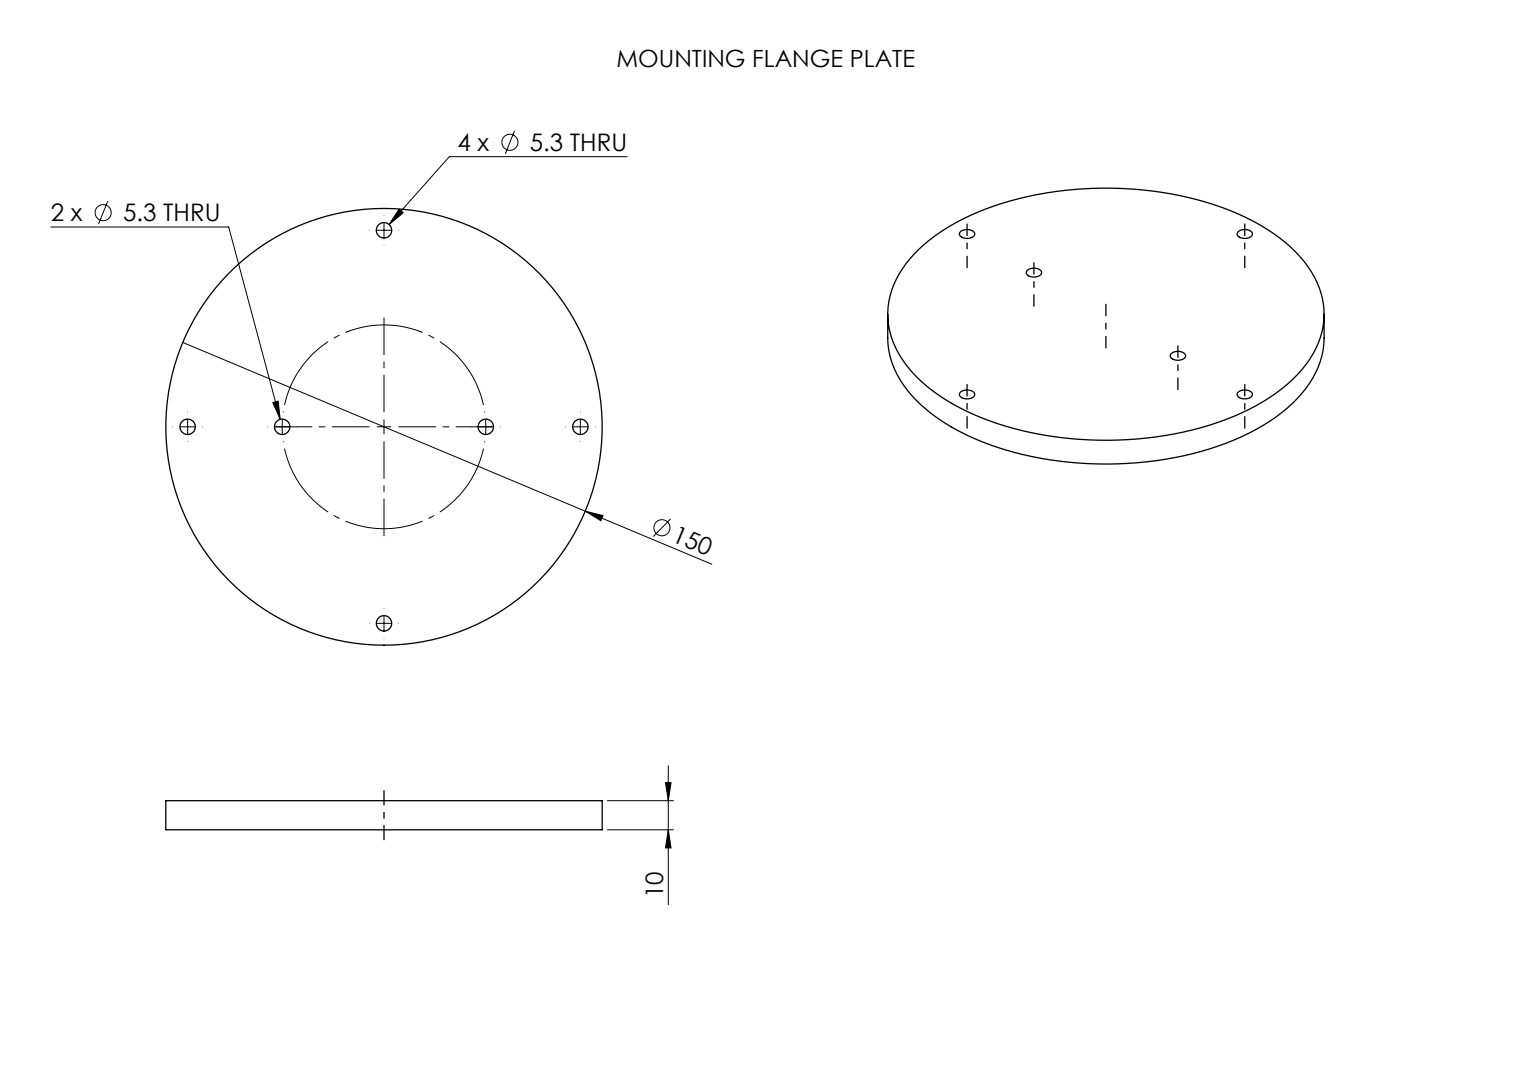
ISO-10303-21;
HEADER;
FILE_DESCRIPTION (('STEP AP214'),
    '1' );
FILE_NAME ('Mounting Flange Plate.step',
    '2026-10-08T13:56:24',
    ( '' ),
    ( '' ),
    'SwSTEP 2.0',
    'SolidWorks 2026',
    '' );
FILE_SCHEMA (( 'AUTOMOTIVE_DESIGN' ));
ENDSEC;

DATA;
#8=CARTESIAN_POINT ( 'NONE',  ( 0.000000000000000000, 50.00000000000000000, -75.00000000000004263 ) ) ;
#37=( NAMED_UNIT ( * ) PLANE_ANGLE_UNIT ( ) SI_UNIT ( $, .RADIAN. ) );
#45=LINE ( 'NONE', #8777, #8712 ) ;
#54=LINE ( 'NONE', #13437, #11247 ) ;
#74=VERTEX_POINT ( 'NONE', #3974 ) ;
#115=ORIENTED_EDGE ( 'NONE', *, *, #5097, .T. ) ;
#180=CIRCLE ( 'NONE', #13308, 2.649999999999985700 ) ;
#186=EDGE_CURVE ( 'NONE', #6462, #4993, #11776, .T. ) ;
#203=CIRCLE ( 'NONE', #1999, 2.649999999999992806 ) ;
#276=ADVANCED_FACE ( 'NONE', ( #4161 ), #12794, .F. ) ;
#288=ORIENTED_EDGE ( 'NONE', *, *, #2102, .T. ) ;
#323=ORIENTED_EDGE ( 'NONE', *, *, #1343, .T. ) ;
#330=ORIENTED_EDGE ( 'NONE', *, *, #5825, .T. ) ;
#378=ORIENTED_EDGE ( 'NONE', *, *, #14411, .F. ) ;
#384=DIRECTION ( 'NONE',  ( -0.000000000000000000, 1.000000000000000000, -0.000000000000000000 ) ) ;
#423=AXIS2_PLACEMENT_3D ( 'NONE', #12972, #1755, #11374 ) ;
#427=DIRECTION ( 'NONE',  ( 0.000000000000000000, 1.000000000000000000, 0.000000000000000000 ) ) ;
#439=ORIENTED_EDGE ( 'NONE', *, *, #14620, .F. ) ;
#514=CARTESIAN_POINT ( 'NONE',  ( 2.143131898507869826E-15, 40.00000000000000000, -64.85000000000002274 ) ) ;
#550=CYLINDRICAL_SURFACE ( 'NONE', #13850, 2.649999999999992806 ) ;
#577=ORIENTED_EDGE ( 'NONE', *, *, #4143, .F. ) ;
#602=CIRCLE ( 'NONE', #5747, 2.649999999999985700 ) ;
#613=DIRECTION ( 'NONE',  ( -0.000000000000000000, 1.000000000000000000, -0.000000000000000000 ) ) ;
#624=CARTESIAN_POINT ( 'NONE',  ( 67.49999999999931788, 50.00000000000000000, 2.081668171172168513E-14 ) ) ;
#663=ORIENTED_EDGE ( 'NONE', *, *, #8419, .F. ) ;
#681=AXIS2_PLACEMENT_3D ( 'NONE', #3435, #9655, #15746 ) ;
#778=DIRECTION ( 'NONE',  ( 0.000000000000000000, 0.000000000000000000, 1.000000000000000000 ) ) ;
#793=DIRECTION ( 'NONE',  ( 0.000000000000000000, 0.000000000000000000, 1.000000000000000000 ) ) ;
#841=DIRECTION ( 'NONE',  ( 0.000000000000000000, 0.000000000000000000, 1.000000000000000000 ) ) ;
#848=DIRECTION ( 'NONE',  ( 0.000000000000000000, 0.000000000000000000, 1.000000000000000000 ) ) ;
#921=CARTESIAN_POINT ( 'NONE',  ( -67.50000000000000000, 40.00000000000000000, 2.649999999999285816 ) ) ;
#934=EDGE_CURVE ( 'NONE', #2513, #13261, #602, .T. ) ;
#952=DIRECTION ( 'NONE',  ( 0.000000000000000000, 1.000000000000000000, 0.000000000000000000 ) ) ;
#988=MECHANICAL_DESIGN_GEOMETRIC_PRESENTATION_REPRESENTATION('',(#3323),#4608);
#1003=CARTESIAN_POINT ( 'NONE',  ( 35.00000000000000000, 50.00000000000000000, 2.649999999999985700 ) ) ;
#1012=DIRECTION ( 'NONE',  ( 0.000000000000000000, 0.000000000000000000, 1.000000000000000000 ) ) ;
#1025=ORIENTED_EDGE ( 'NONE', *, *, #5189, .F. ) ;
#1037=VERTEX_POINT ( 'NONE', #9465 ) ;
#1048=FACE_OUTER_BOUND ( 'NONE', #5833, .T. ) ;
#1071=( LENGTH_UNIT ( ) NAMED_UNIT ( * ) SI_UNIT ( .MILLI., .METRE. ) );
#1118=DIRECTION ( 'NONE',  ( -0.000000000000000000, 1.000000000000000000, -0.000000000000000000 ) ) ;
#1121=DIRECTION ( 'NONE',  ( 0.000000000000000000, -0.000000000000000000, 1.000000000000000000 ) ) ;
#1147=CIRCLE ( 'NONE', #10202, 2.649999999999985700 ) ;
#1152=ORIENTED_EDGE ( 'NONE', *, *, #13038, .F. ) ;
#1188=CIRCLE ( 'NONE', #14094, 2.649999999999985700 ) ;
#1194=EDGE_LOOP ( 'NONE', ( #577, #15095 ) ) ;
#1215=ORIENTED_EDGE ( 'NONE', *, *, #14990, .T. ) ;
#1221=VECTOR ( 'NONE', #2375, 1000.000000000000000 ) ;
#1240=CARTESIAN_POINT ( 'NONE',  ( 2.143131898507869826E-15, 50.00000000000000000, -67.50000000000000000 ) ) ;
#1299=ORIENTED_EDGE ( 'NONE', *, *, #3275, .F. ) ;
#1309=SHAPE_REPRESENTATION_RELATIONSHIP ( 'NONE' , 'NONE' ,  #3049, #6582 ) ;
#1338=DIRECTION ( 'NONE',  ( -0.000000000000000000, 1.000000000000000000, -0.000000000000000000 ) ) ;
#1343=EDGE_CURVE ( 'NONE', #4219, #74, #1876, .T. ) ;
#1369=LINE ( 'NONE', #10033, #13813 ) ;
#1412=EDGE_LOOP ( 'NONE', ( #9601, #5953, #4082, #1598 ) ) ;
#1417=AXIS2_PLACEMENT_3D ( 'NONE', #14635, #4617, #15541 ) ;
#1444=DIRECTION ( 'NONE',  ( -0.000000000000000000, 1.000000000000000000, -0.000000000000000000 ) ) ;
#1557=ADVANCED_FACE ( 'NONE', ( #1841 ), #4363, .F. ) ;
#1598=ORIENTED_EDGE ( 'NONE', *, *, #8419, .T. ) ;
#1624=CARTESIAN_POINT ( 'NONE',  ( -6.765421556309547668E-13, 40.00000000000000000, 67.49999999999930367 ) ) ;
#1658=ADVANCED_FACE ( 'NONE', ( #2550, #7189, #4907, #6041, #9667, #3612, #13379 ), #15756, .T. ) ;
#1679=ORIENTED_EDGE ( 'NONE', *, *, #6309, .F. ) ;
#1699=ORIENTED_EDGE ( 'NONE', *, *, #14620, .T. ) ;
#1709=AXIS2_PLACEMENT_3D ( 'NONE', #7658, #12787, #5294 ) ;
#1711=CARTESIAN_POINT ( 'NONE',  ( 35.00000000000000000, 50.00000000000000000, 2.649999999999992806 ) ) ;
#1726=CYLINDRICAL_SURFACE ( 'NONE', #14159, 2.649999999999992806 ) ;
#1755=DIRECTION ( 'NONE',  ( 0.000000000000000000, 1.000000000000000000, 0.000000000000000000 ) ) ;
#1806=DIRECTION ( 'NONE',  ( 0.000000000000000000, 0.000000000000000000, 1.000000000000000000 ) ) ;
#1841=FACE_OUTER_BOUND ( 'NONE', #15839, .T. ) ;
#1866=AXIS2_PLACEMENT_3D ( 'NONE', #14603, #3524, #3687 ) ;
#1876=CIRCLE ( 'NONE', #3686, 2.649999999999985700 ) ;
#1896=CARTESIAN_POINT ( 'NONE',  ( 35.00000000000000000, 40.00000000000000000, 0.000000000000000000 ) ) ;
#1910=EDGE_LOOP ( 'NONE', ( #3150, #8237 ) ) ;
#1982=VECTOR ( 'NONE', #15334, 1000.000000000000000 ) ;
#1999=AXIS2_PLACEMENT_3D ( 'NONE', #10864, #15807, #4723 ) ;
#2071=VERTEX_POINT ( 'NONE', #4724 ) ;
#2102=EDGE_CURVE ( 'NONE', #12678, #12016, #8834, .T. ) ;
#2181=DIRECTION ( 'NONE',  ( -0.000000000000000000, 1.000000000000000000, -0.000000000000000000 ) ) ;
#2199=( LENGTH_UNIT ( ) NAMED_UNIT ( * ) SI_UNIT ( .MILLI., .METRE. ) );
#2202=AXIS2_PLACEMENT_3D ( 'NONE', #14543, #3463, #3788 ) ;
#2204=ORIENTED_EDGE ( 'NONE', *, *, #4643, .T. ) ;
#2260=CARTESIAN_POINT ( 'NONE',  ( 35.00000000000000000, 40.00000000000000000, 0.000000000000000000 ) ) ;
#2281=EDGE_CURVE ( 'NONE', #15345, #10675, #14755, .T. ) ;
#2289=( NAMED_UNIT ( * ) PLANE_ANGLE_UNIT ( ) SI_UNIT ( $, .RADIAN. ) );
#2375=DIRECTION ( 'NONE',  ( -0.000000000000000000, -1.000000000000000000, -0.000000000000000000 ) ) ;
#2386=CARTESIAN_POINT ( 'NONE',  ( -67.50000000000000000, 50.00000000000000000, 2.649999999999278710 ) ) ;
#2455=ORIENTED_EDGE ( 'NONE', *, *, #8323, .T. ) ;
#2512=( LENGTH_UNIT ( ) NAMED_UNIT ( * ) SI_UNIT ( .MILLI., .METRE. ) );
#2513=VERTEX_POINT ( 'NONE', #13646 ) ;
#2534=ORIENTED_EDGE ( 'NONE', *, *, #8630, .F. ) ;
#2537=CARTESIAN_POINT ( 'NONE',  ( -35.00000000000000000, 50.00000000000000000, -2.649999999999992806 ) ) ;
#2550=FACE_BOUND ( 'NONE', #13651, .T. ) ;
#2561=EDGE_LOOP ( 'NONE', ( #1299, #2455, #1699, #1152 ) ) ;
#2598=( NAMED_UNIT ( * ) SI_UNIT ( $, .STERADIAN. ) SOLID_ANGLE_UNIT ( ) );
#2611=DIRECTION ( 'NONE',  ( -0.000000000000000000, 1.000000000000000000, -0.000000000000000000 ) ) ;
#2689=DIRECTION ( 'NONE',  ( 0.000000000000000000, 0.000000000000000000, 1.000000000000000000 ) ) ;
#2703=ORIENTED_EDGE ( 'NONE', *, *, #11988, .F. ) ;
#2726=DIRECTION ( 'NONE',  ( 0.000000000000000000, 1.000000000000000000, 0.000000000000000000 ) ) ;
#2738=DIRECTION ( 'NONE',  ( -0.000000000000000000, 1.000000000000000000, -0.000000000000000000 ) ) ;
#2811=ORIENTED_EDGE ( 'NONE', *, *, #6309, .T. ) ;
#2835=ORIENTED_EDGE ( 'NONE', *, *, #5189, .T. ) ;
#2841=DIRECTION ( 'NONE',  ( -0.000000000000000000, 1.000000000000000000, -0.000000000000000000 ) ) ;
#2873=APPLICATION_CONTEXT ( 'automotive_design' ) ;
#2874=FACE_OUTER_BOUND ( 'NONE', #3579, .T. ) ;
#2960=CYLINDRICAL_SURFACE ( 'NONE', #681, 75.00000000000004263 ) ;
#3021=VECTOR ( 'NONE', #13757, 1000.000000000000000 ) ;
#3049=SHAPE_REPRESENTATION ( 'Mounting Flange Plate', ( #3223 ), #15373 ) ;
#3055=ORIENTED_EDGE ( 'NONE', *, *, #4930, .F. ) ;
#3118=VERTEX_POINT ( 'NONE', #10334 ) ;
#3138=CARTESIAN_POINT ( 'NONE',  ( 67.49999999999931788, 40.00000000000000000, 2.081668171172168513E-14 ) ) ;
#3141=DIRECTION ( 'NONE',  ( 0.000000000000000000, 0.000000000000000000, 1.000000000000000000 ) ) ;
#3150=ORIENTED_EDGE ( 'NONE', *, *, #15289, .T. ) ;
#3191=VERTEX_POINT ( 'NONE', #5708 ) ;
#3223=AXIS2_PLACEMENT_3D ( 'NONE', #11897, #11972, #4638 ) ;
#3248=AXIS2_PLACEMENT_3D ( 'NONE', #15818, #3291, #793 ) ;
#3253=AXIS2_PLACEMENT_3D ( 'NONE', #3138, #8007, #14453 ) ;
#3266=CARTESIAN_POINT ( 'NONE',  ( -35.00000000000000000, 50.00000000000000000, 2.649999999999985700 ) ) ;
#3270=CYLINDRICAL_SURFACE ( 'NONE', #6972, 2.649999999999985700 ) ;
#3275=EDGE_CURVE ( 'NONE', #10300, #9472, #15960, .T. ) ;
#3291=DIRECTION ( 'NONE',  ( -0.000000000000000000, 1.000000000000000000, -0.000000000000000000 ) ) ;
#3323=STYLED_ITEM ( 'NONE', ( #14492 ), #9475 ) ;
#3435=CARTESIAN_POINT ( 'NONE',  ( 0.000000000000000000, 50.00000000000000000, 0.000000000000000000 ) ) ;
#3463=DIRECTION ( 'NONE',  ( -0.000000000000000000, 1.000000000000000000, -0.000000000000000000 ) ) ;
#3472=CIRCLE ( 'NONE', #10961, 75.00000000000004263 ) ;
#3524=DIRECTION ( 'NONE',  ( 0.000000000000000000, 1.000000000000000000, 0.000000000000000000 ) ) ;
#3543=CARTESIAN_POINT ( 'NONE',  ( -67.50000000000000000, 50.00000000000000000, 2.649999999999285816 ) ) ;
#3579=EDGE_LOOP ( 'NONE', ( #10493, #4203, #6813, #9254 ) ) ;
#3580=CARTESIAN_POINT ( 'NONE',  ( -6.765421556309547668E-13, 50.00000000000000000, 70.14999999999929514 ) ) ;
#3609=APPLICATION_CONTEXT ( 'automotive_design' ) ;
#3612=FACE_BOUND ( 'NONE', #11613, .T. ) ;
#3641=CARTESIAN_POINT ( 'NONE',  ( 9.184850993605153466E-15, 50.00000000000000000, 75.00000000000004263 ) ) ;
#3651=AXIS2_PLACEMENT_3D ( 'NONE', #2260, #10529, #9467 ) ;
#3657=SURFACE_STYLE_FILL_AREA ( #13668 ) ;
#3686=AXIS2_PLACEMENT_3D ( 'NONE', #6471, #1444, #10349 ) ;
#3687=DIRECTION ( 'NONE',  ( 0.000000000000000000, -0.000000000000000000, 1.000000000000000000 ) ) ;
#3703=ORIENTED_EDGE ( 'NONE', *, *, #14672, .F. ) ;
#3706=FACE_BOUND ( 'NONE', #13137, .T. ) ;
#3732=SURFACE_SIDE_STYLE ('',( #3657 ) ) ;
#3745=DIRECTION ( 'NONE',  ( -0.000000000000000000, 1.000000000000000000, -0.000000000000000000 ) ) ;
#3788=DIRECTION ( 'NONE',  ( 0.000000000000000000, 0.000000000000000000, 1.000000000000000000 ) ) ;
#3791=PLANE ( 'NONE',  #15961 ) ;
#3795=ADVANCED_FACE ( 'NONE', ( #12612 ), #6330, .F. ) ;
#3821=FILL_AREA_STYLE_COLOUR ( '', #6625 ) ;
#3898=DIRECTION ( 'NONE',  ( 0.000000000000000000, 1.000000000000000000, 0.000000000000000000 ) ) ;
#3923=DIRECTION ( 'NONE',  ( 0.000000000000000000, 0.000000000000000000, 1.000000000000000000 ) ) ;
#3964=CARTESIAN_POINT ( 'NONE',  ( 0.000000000000000000, 50.00000000000000000, 0.000000000000000000 ) ) ;
#3974=CARTESIAN_POINT ( 'NONE',  ( 2.143131898507869826E-15, 50.00000000000000000, -64.85000000000002274 ) ) ;
#3981=CARTESIAN_POINT ( 'NONE',  ( 67.49999999999931788, 50.00000000000000000, 2.650000000000013678 ) ) ;
#4019=EDGE_CURVE ( 'NONE', #10675, #15938, #5597, .T. ) ;
#4023=CIRCLE ( 'NONE', #423, 2.649999999999992806 ) ;
#4030=CARTESIAN_POINT ( 'NONE',  ( -67.50000000000000000, 50.00000000000000000, -7.070249711157346244E-13 ) ) ;
#4041=CIRCLE ( 'NONE', #9713, 2.649999999999985700 ) ;
#4082=ORIENTED_EDGE ( 'NONE', *, *, #13038, .T. ) ;
#4087=DIRECTION ( 'NONE',  ( 0.000000000000000000, 0.000000000000000000, 1.000000000000000000 ) ) ;
#4122=ORIENTED_EDGE ( 'NONE', *, *, #4947, .F. ) ;
#4143=EDGE_CURVE ( 'NONE', #2071, #14412, #180, .T. ) ;
#4161=FACE_OUTER_BOUND ( 'NONE', #10744, .T. ) ;
#4203=ORIENTED_EDGE ( 'NONE', *, *, #15548, .T. ) ;
#4219=VERTEX_POINT ( 'NONE', #4478 ) ;
#4247=DIRECTION ( 'NONE',  ( 0.000000000000000000, 0.000000000000000000, 1.000000000000000000 ) ) ;
#4259=ORIENTED_EDGE ( 'NONE', *, *, #186, .F. ) ;
#4335=CIRCLE ( 'NONE', #10006, 2.649999999999985700 ) ;
#4342=CARTESIAN_POINT ( 'NONE',  ( 35.00000000000000000, 50.00000000000000000, -2.649999999999992806 ) ) ;
#4363=CYLINDRICAL_SURFACE ( 'NONE', #7560, 2.649999999999985700 ) ;
#4440=VERTEX_POINT ( 'NONE', #2386 ) ;
#4443=ADVANCED_FACE ( 'NONE', ( #2874 ), #11200, .F. ) ;
#4450=ORIENTED_EDGE ( 'NONE', *, *, #7947, .T. ) ;
#4478=CARTESIAN_POINT ( 'NONE',  ( 2.467663300281918126E-15, 50.00000000000000000, -70.14999999999999147 ) ) ;
#4560=FACE_OUTER_BOUND ( 'NONE', #10471, .T. ) ;
#4569=VECTOR ( 'NONE', #14181, 1000.000000000000000 ) ;
#4595=LINE ( 'NONE', #14384, #1221 ) ;
#4607=VECTOR ( 'NONE', #12069, 1000.000000000000000 ) ;
#4608=( GEOMETRIC_REPRESENTATION_CONTEXT ( 3 ) GLOBAL_UNCERTAINTY_ASSIGNED_CONTEXT ( ( #14034 ) ) GLOBAL_UNIT_ASSIGNED_CONTEXT ( ( #2199, #15793, #10932 ) ) REPRESENTATION_CONTEXT ( 'NONE', 'WORKASPACE' ) );
#4617=DIRECTION ( 'NONE',  ( -0.000000000000000000, 1.000000000000000000, -0.000000000000000000 ) ) ;
#4638=DIRECTION ( 'NONE',  ( 1.000000000000000000, 0.000000000000000000, 0.000000000000000000 ) ) ;
#4643=EDGE_CURVE ( 'NONE', #6800, #6071, #9114, .T. ) ;
#4645=EDGE_LOOP ( 'NONE', ( #7116, #4799, #13900, #5382 ) ) ;
#4661=ADVANCED_FACE ( 'NONE', ( #13042 ), #550, .F. ) ;
#4694=ORIENTED_EDGE ( 'NONE', *, *, #4947, .T. ) ;
#4723=DIRECTION ( 'NONE',  ( 0.000000000000000000, 0.000000000000000000, 1.000000000000000000 ) ) ;
#4724=CARTESIAN_POINT ( 'NONE',  ( -6.765421556309547668E-13, 50.00000000000000000, 70.14999999999929514 ) ) ;
#4726=CARTESIAN_POINT ( 'NONE',  ( 2.467663300281917732E-15, 50.00000000000000000, -70.14999999999999147 ) ) ;
#4763=LINE ( 'NONE', #3543, #11243 ) ;
#4772=DIRECTION ( 'NONE',  ( 0.000000000000000000, 0.000000000000000000, 1.000000000000000000 ) ) ;
#4799=ORIENTED_EDGE ( 'NONE', *, *, #5413, .T. ) ;
#4821=EDGE_CURVE ( 'NONE', #3191, #6800, #5082, .T. ) ;
#4861=DIRECTION ( 'NONE',  ( -0.000000000000000000, 1.000000000000000000, -0.000000000000000000 ) ) ;
#4864=EDGE_LOOP ( 'NONE', ( #8155, #13074, #2811, #5258 ) ) ;
#4881=CARTESIAN_POINT ( 'NONE',  ( 9.184850993605153466E-15, 40.00000000000000000, 75.00000000000004263 ) ) ;
#4907=FACE_BOUND ( 'NONE', #8075, .T. ) ;
#4921=CARTESIAN_POINT ( 'NONE',  ( 67.49999999999931788, 50.00000000000000000, 2.650000000000006573 ) ) ;
#4923=EDGE_LOOP ( 'NONE', ( #8098, #8858 ) ) ;
#4930=EDGE_CURVE ( 'NONE', #6800, #3191, #203, .T. ) ;
#4947=EDGE_CURVE ( 'NONE', #74, #4219, #10273, .T. ) ;
#4950=LINE ( 'NONE', #3580, #7713 ) ;
#4993=VERTEX_POINT ( 'NONE', #14823 ) ;
#5029=( GEOMETRIC_REPRESENTATION_CONTEXT ( 3 ) GLOBAL_UNCERTAINTY_ASSIGNED_CONTEXT ( ( #12385 ) ) GLOBAL_UNIT_ASSIGNED_CONTEXT ( ( #2512, #2289, #2598 ) ) REPRESENTATION_CONTEXT ( 'NONE', 'WORKASPACE' ) );
#5044=DIRECTION ( 'NONE',  ( -0.000000000000000000, 1.000000000000000000, -0.000000000000000000 ) ) ;
#5062=EDGE_CURVE ( 'NONE', #12678, #74, #45, .T. ) ;
#5082=CIRCLE ( 'NONE', #8970, 2.649999999999992806 ) ;
#5097=EDGE_CURVE ( 'NONE', #6462, #11470, #13678, .T. ) ;
#5107=AXIS2_PLACEMENT_3D ( 'NONE', #10299, #2841, #9003 ) ;
#5122=CARTESIAN_POINT ( 'NONE',  ( 35.00000000000000000, 40.00000000000000000, 2.649999999999992806 ) ) ;
#5134=CARTESIAN_POINT ( 'NONE',  ( -35.00000000000000000, 50.00000000000000000, 0.000000000000000000 ) ) ;
#5189=EDGE_CURVE ( 'NONE', #9703, #1037, #12700, .T. ) ;
#5235=ORIENTED_EDGE ( 'NONE', *, *, #14818, .T. ) ;
#5258=ORIENTED_EDGE ( 'NONE', *, *, #4143, .T. ) ;
#5294=DIRECTION ( 'NONE',  ( 0.000000000000000000, 0.000000000000000000, 1.000000000000000000 ) ) ;
#5364=AXIS2_PLACEMENT_3D ( 'NONE', #1240, #3745, #2689 ) ;
#5382=ORIENTED_EDGE ( 'NONE', *, *, #4019, .F. ) ;
#5413=EDGE_CURVE ( 'NONE', #15345, #3118, #5551, .T. ) ;
#5432=DIRECTION ( 'NONE',  ( 0.000000000000000000, 0.000000000000000000, -1.000000000000000000 ) ) ;
#5442=ORIENTED_EDGE ( 'NONE', *, *, #14990, .F. ) ;
#5454=CARTESIAN_POINT ( 'NONE',  ( -67.50000000000000000, 50.00000000000000000, -7.070249711157346244E-13 ) ) ;
#5551=LINE ( 'NONE', #4342, #6910 ) ;
#5597=LINE ( 'NONE', #1711, #10011 ) ;
#5704=DIRECTION ( 'NONE',  ( -0.000000000000000000, 1.000000000000000000, -0.000000000000000000 ) ) ;
#5708=CARTESIAN_POINT ( 'NONE',  ( -35.00000000000000000, 40.00000000000000000, -2.649999999999992806 ) ) ;
#5747=AXIS2_PLACEMENT_3D ( 'NONE', #1624, #427, #15219 ) ;
#5766=CARTESIAN_POINT ( 'NONE',  ( -6.765421556309547668E-13, 50.00000000000000000, 67.49999999999930367 ) ) ;
#5768=ORIENTED_EDGE ( 'NONE', *, *, #14393, .F. ) ;
#5796=CIRCLE ( 'NONE', #14833, 2.649999999999992806 ) ;
#5825=EDGE_CURVE ( 'NONE', #14592, #10616, #4595, .T. ) ;
#5833=EDGE_LOOP ( 'NONE', ( #14308, #2703 ) ) ;
#5859=AXIS2_PLACEMENT_3D ( 'NONE', #3964, #10118, #5432 ) ;
#5865=LINE ( 'NONE', #4726, #4607 ) ;
#5895=AXIS2_PLACEMENT_3D ( 'NONE', #8233, #8070, #13129 ) ;
#5920=ORIENTED_EDGE ( 'NONE', *, *, #14818, .F. ) ;
#5935=EDGE_LOOP ( 'NONE', ( #12559, #8528 ) ) ;
#5936=DIRECTION ( 'NONE',  ( -0.000000000000000000, 1.000000000000000000, -0.000000000000000000 ) ) ;
#5953=ORIENTED_EDGE ( 'NONE', *, *, #15289, .F. ) ;
#5980=DIRECTION ( 'NONE',  ( 0.000000000000000000, 0.000000000000000000, 1.000000000000000000 ) ) ;
#6009=PRODUCT_DEFINITION ( 'UNKNOWN', '', #6905, #6432 ) ;
#6041=FACE_BOUND ( 'NONE', #8449, .T. ) ;
#6059=CARTESIAN_POINT ( 'NONE',  ( -6.765421556309547668E-13, 50.00000000000000000, 67.49999999999930367 ) ) ;
#6071=VERTEX_POINT ( 'NONE', #3266 ) ;
#6113=ORIENTED_EDGE ( 'NONE', *, *, #11650, .T. ) ;
#6229=FACE_BOUND ( 'NONE', #11318, .T. ) ;
#6309=EDGE_CURVE ( 'NONE', #2513, #2071, #4950, .T. ) ;
#6312=DIRECTION ( 'NONE',  ( -0.000000000000000000, 1.000000000000000000, -0.000000000000000000 ) ) ;
#6330=CYLINDRICAL_SURFACE ( 'NONE', #5107, 2.649999999999985700 ) ;
#6337=DIRECTION ( 'NONE',  ( 0.000000000000000000, 0.000000000000000000, 1.000000000000000000 ) ) ;
#6355=LINE ( 'NONE', #2537, #15909 ) ;
#6398=EDGE_LOOP ( 'NONE', ( #13187, #3055, #2204, #4450 ) ) ;
#6407=FACE_OUTER_BOUND ( 'NONE', #15268, .T. ) ;
#6432=PRODUCT_DEFINITION_CONTEXT ( 'detailed design', #3609, 'design' ) ;
#6462=VERTEX_POINT ( 'NONE', #9960 ) ;
#6471=CARTESIAN_POINT ( 'NONE',  ( 2.143131898507869826E-15, 50.00000000000000000, -67.50000000000000000 ) ) ;
#6562=ADVANCED_FACE ( 'NONE', ( #9777, #6229, #3706, #9929, #12352, #7209, #1048 ), #3791, .F. ) ;
#6582=ADVANCED_BREP_SHAPE_REPRESENTATION ( '', ( #9475, #3223 ), #15373 ) ;
#6625=COLOUR_RGB ( '', 0.09019608, 0.27058824, 0.51372549) ;
#6687=EDGE_LOOP ( 'NONE', ( #10153, #13602, #7741, #4694 ) ) ;
#6710=DIRECTION ( 'NONE',  ( 0.000000000000000000, 0.000000000000000000, 1.000000000000000000 ) ) ;
#6800=VERTEX_POINT ( 'NONE', #11106 ) ;
#6813=ORIENTED_EDGE ( 'NONE', *, *, #12208, .T. ) ;
#6905=PRODUCT_DEFINITION_FORMATION_WITH_SPECIFIED_SOURCE ( 'ANY', '', #8502, .NOT_KNOWN. ) ;
#6910=VECTOR ( 'NONE', #10576, 1000.000000000000000 ) ;
#6972=AXIS2_PLACEMENT_3D ( 'NONE', #15489, #5936, #848 ) ;
#7036=CARTESIAN_POINT ( 'NONE',  ( 0.000000000000000000, 50.00000000000000000, 0.000000000000000000 ) ) ;
#7067=PRODUCT_DEFINITION_SHAPE ( 'NONE', 'NONE',  #6009 ) ;
#7116=ORIENTED_EDGE ( 'NONE', *, *, #2281, .F. ) ;
#7189=FACE_BOUND ( 'NONE', #4923, .T. ) ;
#7209=FACE_BOUND ( 'NONE', #5935, .T. ) ;
#7233=SURFACE_STYLE_USAGE ( .BOTH. , #12207 ) ;
#7325=DIRECTION ( 'NONE',  ( -0.000000000000000000, 1.000000000000000000, -0.000000000000000000 ) ) ;
#7560=AXIS2_PLACEMENT_3D ( 'NONE', #15591, #9298, #3141 ) ;
#7638=CARTESIAN_POINT ( 'NONE',  ( 67.49999999999931788, 40.00000000000000000, 2.081668171172168513E-14 ) ) ;
#7658=CARTESIAN_POINT ( 'NONE',  ( 0.000000000000000000, 50.00000000000000000, 0.000000000000000000 ) ) ;
#7707=AXIS2_PLACEMENT_3D ( 'NONE', #15447, #15359, #15678 ) ;
#7713=VECTOR ( 'NONE', #9878, 1000.000000000000000 ) ;
#7741=ORIENTED_EDGE ( 'NONE', *, *, #5062, .T. ) ;
#7859=ORIENTED_EDGE ( 'NONE', *, *, #4019, .T. ) ;
#7861=EDGE_CURVE ( 'NONE', #12016, #4219, #5865, .T. ) ;
#7917=FACE_OUTER_BOUND ( 'NONE', #4864, .T. ) ;
#7943=VERTEX_POINT ( 'NONE', #9816 ) ;
#7947=EDGE_CURVE ( 'NONE', #6071, #15584, #9514, .T. ) ;
#7964=COLOUR_RGB ( '', 0.09019608, 0.27058824, 0.51372549) ;
#8007=DIRECTION ( 'NONE',  ( 0.000000000000000000, 1.000000000000000000, 0.000000000000000000 ) ) ;
#8035=SHAPE_DEFINITION_REPRESENTATION ( #7067, #3049 ) ;
#8070=DIRECTION ( 'NONE',  ( 0.000000000000000000, 1.000000000000000000, 0.000000000000000000 ) ) ;
#8075=EDGE_LOOP ( 'NONE', ( #4122, #13632 ) ) ;
#8098=ORIENTED_EDGE ( 'NONE', *, *, #7947, .F. ) ;
#8143=AXIS2_PLACEMENT_3D ( 'NONE', #8515, #4861, #8586 ) ;
#8153=EDGE_LOOP ( 'NONE', ( #11271, #6113 ) ) ;
#8154=FACE_OUTER_BOUND ( 'NONE', #4645, .T. ) ;
#8155=ORIENTED_EDGE ( 'NONE', *, *, #15691, .F. ) ;
#8195=ORIENTED_EDGE ( 'NONE', *, *, #15814, .F. ) ;
#8233=CARTESIAN_POINT ( 'NONE',  ( -67.50000000000000000, 40.00000000000000000, -7.070249711157346244E-13 ) ) ;
#8237=ORIENTED_EDGE ( 'NONE', *, *, #3275, .T. ) ;
#8323=EDGE_CURVE ( 'NONE', #10300, #13915, #11386, .T. ) ;
#8406=CIRCLE ( 'NONE', #1709, 75.00000000000004263 ) ;
#8419=EDGE_CURVE ( 'NONE', #4440, #13915, #4335, .T. ) ;
#8449=EDGE_LOOP ( 'NONE', ( #663, #439 ) ) ;
#8476=CARTESIAN_POINT ( 'NONE',  ( 0.000000000000000000, 40.00000000000000000, 0.000000000000000000 ) ) ;
#8499=DIRECTION ( 'NONE',  ( 0.000000000000000000, 0.000000000000000000, 1.000000000000000000 ) ) ;
#8502=PRODUCT ( 'Mounting Flange Plate', 'Mounting Flange Plate', '', ( #12851 ) ) ;
#8515=CARTESIAN_POINT ( 'NONE',  ( -67.50000000000000000, 50.00000000000000000, -7.070249711157346244E-13 ) ) ;
#8527=SURFACE_STYLE_FILL_AREA ( #9563 ) ;
#8528=ORIENTED_EDGE ( 'NONE', *, *, #13280, .T. ) ;
#8552=ORIENTED_EDGE ( 'NONE', *, *, #2281, .T. ) ;
#8568=ORIENTED_EDGE ( 'NONE', *, *, #13110, .T. ) ;
#8586=DIRECTION ( 'NONE',  ( 0.000000000000000000, 0.000000000000000000, 1.000000000000000000 ) ) ;
#8615=DIRECTION ( 'NONE',  ( 0.000000000000000000, 0.000000000000000000, 1.000000000000000000 ) ) ;
#8630=EDGE_CURVE ( 'NONE', #15938, #3118, #14653, .T. ) ;
#8712=VECTOR ( 'NONE', #5044, 1000.000000000000000 ) ;
#8752=AXIS2_PLACEMENT_3D ( 'NONE', #5134, #2611, #12386 ) ;
#8777=CARTESIAN_POINT ( 'NONE',  ( 2.143131898507869826E-15, 50.00000000000000000, -64.85000000000002274 ) ) ;
#8821=DIRECTION ( 'NONE',  ( 0.000000000000000000, 0.000000000000000000, 1.000000000000000000 ) ) ;
#8826=ORIENTED_EDGE ( 'NONE', *, *, #13280, .F. ) ;
#8834=CIRCLE ( 'NONE', #10638, 2.649999999999985700 ) ;
#8845=EDGE_LOOP ( 'NONE', ( #11934, #1215 ) ) ;
#8858=ORIENTED_EDGE ( 'NONE', *, *, #12208, .F. ) ;
#8924=CIRCLE ( 'NONE', #14324, 2.649999999999985700 ) ;
#8950=AXIS2_PLACEMENT_3D ( 'NONE', #10343, #15433, #6710 ) ;
#8954=DIRECTION ( 'NONE',  ( 0.000000000000000000, 0.000000000000000000, 1.000000000000000000 ) ) ;
#8970=AXIS2_PLACEMENT_3D ( 'NONE', #13504, #11909, #1012 ) ;
#9003=DIRECTION ( 'NONE',  ( 0.000000000000000000, 0.000000000000000000, 1.000000000000000000 ) ) ;
#9094=CARTESIAN_POINT ( 'NONE',  ( 0.000000000000000000, 50.00000000000000000, -75.00000000000004263 ) ) ;
#9114=LINE ( 'NONE', #12801, #1982 ) ;
#9188=CIRCLE ( 'NONE', #11238, 75.00000000000004263 ) ;
#9254=ORIENTED_EDGE ( 'NONE', *, *, #4643, .F. ) ;
#9298=DIRECTION ( 'NONE',  ( -0.000000000000000000, 1.000000000000000000, -0.000000000000000000 ) ) ;
#9354=ADVANCED_FACE ( 'NONE', ( #9408 ), #1726, .F. ) ;
#9408=FACE_OUTER_BOUND ( 'NONE', #2561, .T. ) ;
#9421=DIRECTION ( 'NONE',  ( -0.000000000000000000, 1.000000000000000000, -0.000000000000000000 ) ) ;
#9465=CARTESIAN_POINT ( 'NONE',  ( 0.000000000000000000, 40.00000000000000000, -75.00000000000004263 ) ) ;
#9467=DIRECTION ( 'NONE',  ( 0.000000000000000000, 0.000000000000000000, 1.000000000000000000 ) ) ;
#9472=VERTEX_POINT ( 'NONE', #921 ) ;
#9475=MANIFOLD_SOLID_BREP ( 'CirPattern1', #12026 ) ;
#9514=CIRCLE ( 'NONE', #8752, 2.649999999999985700 ) ;
#9523=CARTESIAN_POINT ( 'NONE',  ( -6.762176242291807225E-13, 40.00000000000000000, 64.84999999999932641 ) ) ;
#9563=FILL_AREA_STYLE ('',( #11016 ) ) ;
#9589=DIRECTION ( 'NONE',  ( 0.000000000000000000, 0.000000000000000000, 1.000000000000000000 ) ) ;
#9601=ORIENTED_EDGE ( 'NONE', *, *, #8323, .F. ) ;
#9607=CYLINDRICAL_SURFACE ( 'NONE', #2202, 2.649999999999992806 ) ;
#9655=DIRECTION ( 'NONE',  ( -0.000000000000000000, -1.000000000000000000, -0.000000000000000000 ) ) ;
#9667=FACE_BOUND ( 'NONE', #1194, .T. ) ;
#9677=DIRECTION ( 'NONE',  ( 0.000000000000000000, 0.000000000000000000, 1.000000000000000000 ) ) ;
#9684=DIRECTION ( 'NONE',  ( -0.000000000000000000, 1.000000000000000000, -0.000000000000000000 ) ) ;
#9703=VERTEX_POINT ( 'NONE', #8 ) ;
#9713=AXIS2_PLACEMENT_3D ( 'NONE', #624, #9421, #778 ) ;
#9777=FACE_BOUND ( 'NONE', #12736, .T. ) ;
#9815=CARTESIAN_POINT ( 'NONE',  ( 2.143131898507869826E-15, 40.00000000000000000, -67.50000000000000000 ) ) ;
#9816=CARTESIAN_POINT ( 'NONE',  ( 67.49999999999931788, 50.00000000000000000, -2.649999999999964828 ) ) ;
#9878=DIRECTION ( 'NONE',  ( -0.000000000000000000, 1.000000000000000000, -0.000000000000000000 ) ) ;
#9904=DIRECTION ( 'NONE',  ( 0.000000000000000000, 0.000000000000000000, 1.000000000000000000 ) ) ;
#9929=FACE_BOUND ( 'NONE', #1910, .T. ) ;
#9960=CARTESIAN_POINT ( 'NONE',  ( 67.49999999999931788, 40.00000000000000000, 2.650000000000013678 ) ) ;
#9997=FACE_OUTER_BOUND ( 'NONE', #1412, .T. ) ;
#9998=CARTESIAN_POINT ( 'NONE',  ( -35.00000000000000000, 50.00000000000000000, 0.000000000000000000 ) ) ;
#10006=AXIS2_PLACEMENT_3D ( 'NONE', #4030, #6312, #8821 ) ;
#10011=VECTOR ( 'NONE', #11567, 1000.000000000000000 ) ;
#10033=CARTESIAN_POINT ( 'NONE',  ( 67.49999999999931788, 50.00000000000000000, -2.649999999999971934 ) ) ;
#10118=DIRECTION ( 'NONE',  ( -0.000000000000000000, -1.000000000000000000, -0.000000000000000000 ) ) ;
#10153=ORIENTED_EDGE ( 'NONE', *, *, #7861, .F. ) ;
#10202=AXIS2_PLACEMENT_3D ( 'NONE', #13406, #10999, #841 ) ;
#10273=CIRCLE ( 'NONE', #5364, 2.649999999999985700 ) ;
#10288=CYLINDRICAL_SURFACE ( 'NONE', #5859, 75.00000000000004263 ) ;
#10299=CARTESIAN_POINT ( 'NONE',  ( 2.143131898507869826E-15, 50.00000000000000000, -67.50000000000000000 ) ) ;
#10300=VERTEX_POINT ( 'NONE', #14861 ) ;
#10334=CARTESIAN_POINT ( 'NONE',  ( 35.00000000000000000, 50.00000000000000000, -2.649999999999985700 ) ) ;
#10343=CARTESIAN_POINT ( 'NONE',  ( -6.765421556309547668E-13, 50.00000000000000000, 67.49999999999930367 ) ) ;
#10349=DIRECTION ( 'NONE',  ( 0.000000000000000000, 0.000000000000000000, 1.000000000000000000 ) ) ;
#10471=EDGE_LOOP ( 'NONE', ( #15782, #11881, #8568, #1679 ) ) ;
#10486=ADVANCED_FACE ( 'NONE', ( #4560 ), #3270, .F. ) ;
#10493=ORIENTED_EDGE ( 'NONE', *, *, #4821, .F. ) ;
#10496=ORIENTED_EDGE ( 'NONE', *, *, #4821, .T. ) ;
#10529=DIRECTION ( 'NONE',  ( 0.000000000000000000, 1.000000000000000000, 0.000000000000000000 ) ) ;
#10576=DIRECTION ( 'NONE',  ( -0.000000000000000000, 1.000000000000000000, -0.000000000000000000 ) ) ;
#10616=VERTEX_POINT ( 'NONE', #4881 ) ;
#10638=AXIS2_PLACEMENT_3D ( 'NONE', #9815, #14744, #8615 ) ;
#10675=VERTEX_POINT ( 'NONE', #5122 ) ;
#10708=AXIS2_PLACEMENT_3D ( 'NONE', #13697, #384, #4087 ) ;
#10744=EDGE_LOOP ( 'NONE', ( #5920, #4259, #115, #14639 ) ) ;
#10846=ORIENTED_EDGE ( 'NONE', *, *, #7861, .T. ) ;
#10864=CARTESIAN_POINT ( 'NONE',  ( -35.00000000000000000, 40.00000000000000000, 0.000000000000000000 ) ) ;
#10903=CARTESIAN_POINT ( 'NONE',  ( 35.00000000000000000, 50.00000000000000000, 0.000000000000000000 ) ) ;
#10932=( NAMED_UNIT ( * ) SI_UNIT ( $, .STERADIAN. ) SOLID_ANGLE_UNIT ( ) );
#10958=DIRECTION ( 'NONE',  ( 0.000000000000000000, 1.000000000000000000, 0.000000000000000000 ) ) ;
#10961=AXIS2_PLACEMENT_3D ( 'NONE', #8476, #952, #9904 ) ;
#10999=DIRECTION ( 'NONE',  ( 0.000000000000000000, 1.000000000000000000, 0.000000000000000000 ) ) ;
#11007=AXIS2_PLACEMENT_3D ( 'NONE', #7638, #3898, #6337 ) ;
#11016=FILL_AREA_STYLE_COLOUR ( '', #7964 ) ;
#11106=CARTESIAN_POINT ( 'NONE',  ( -35.00000000000000000, 40.00000000000000000, 2.649999999999992806 ) ) ;
#11122=DIRECTION ( 'NONE',  ( -0.000000000000000000, 1.000000000000000000, -0.000000000000000000 ) ) ;
#11143=CARTESIAN_POINT ( 'NONE',  ( 0.000000000000000000, 40.00000000000000000, 0.000000000000000000 ) ) ;
#11200=CYLINDRICAL_SURFACE ( 'NONE', #15933, 2.649999999999992806 ) ;
#11217=DIRECTION ( 'NONE',  ( 0.000000000000000000, 0.000000000000000000, 1.000000000000000000 ) ) ;
#11238=AXIS2_PLACEMENT_3D ( 'NONE', #7036, #15682, #9677 ) ;
#11243=VECTOR ( 'NONE', #12260, 1000.000000000000000 ) ;
#11247=VECTOR ( 'NONE', #7325, 1000.000000000000000 ) ;
#11265=UNCERTAINTY_MEASURE_WITH_UNIT (LENGTH_MEASURE( 1.000000000000000082E-05 ), #1071, 'distance_accuracy_value', 'NONE');
#11271=ORIENTED_EDGE ( 'NONE', *, *, #934, .T. ) ;
#11318=EDGE_LOOP ( 'NONE', ( #12275, #10496 ) ) ;
#11374=DIRECTION ( 'NONE',  ( 0.000000000000000000, 0.000000000000000000, 1.000000000000000000 ) ) ;
#11386=LINE ( 'NONE', #13722, #11545 ) ;
#11470=VERTEX_POINT ( 'NONE', #4921 ) ;
#11498=CIRCLE ( 'NONE', #14870, 75.00000000000004263 ) ;
#11545=VECTOR ( 'NONE', #2738, 1000.000000000000000 ) ;
#11554=ORIENTED_EDGE ( 'NONE', *, *, #14672, .T. ) ;
#11567=DIRECTION ( 'NONE',  ( -0.000000000000000000, 1.000000000000000000, -0.000000000000000000 ) ) ;
#11613=EDGE_LOOP ( 'NONE', ( #378, #15365 ) ) ;
#11650=EDGE_CURVE ( 'NONE', #13261, #2513, #1188, .T. ) ;
#11750=AXIS2_PLACEMENT_3D ( 'NONE', #6059, #9684, #8499 ) ;
#11776=CIRCLE ( 'NONE', #11007, 2.649999999999992806 ) ;
#11821=DIRECTION ( 'NONE',  ( 0.000000000000000000, 0.000000000000000000, 1.000000000000000000 ) ) ;
#11845=CYLINDRICAL_SURFACE ( 'NONE', #3248, 2.649999999999992806 ) ;
#11881=ORIENTED_EDGE ( 'NONE', *, *, #15691, .T. ) ;
#11897=CARTESIAN_POINT ( 'NONE',  ( 0.000000000000000000, 0.000000000000000000, 0.000000000000000000 ) ) ;
#11903=ADVANCED_FACE ( 'NONE', ( #7917 ), #12818, .F. ) ;
#11909=DIRECTION ( 'NONE',  ( 0.000000000000000000, 1.000000000000000000, 0.000000000000000000 ) ) ;
#11934=ORIENTED_EDGE ( 'NONE', *, *, #15814, .T. ) ;
#11972=DIRECTION ( 'NONE',  ( 0.000000000000000000, 0.000000000000000000, 1.000000000000000000 ) ) ;
#11980=MECHANICAL_DESIGN_GEOMETRIC_PRESENTATION_REPRESENTATION('',(#14323),#5029);
#11988=EDGE_CURVE ( 'NONE', #10616, #1037, #11498, .T. ) ;
#12003=AXIS2_PLACEMENT_3D ( 'NONE', #10903, #1118, #5980 ) ;
#12016=VERTEX_POINT ( 'NONE', #13523 ) ;
#12026=CLOSED_SHELL ( 'NONE', ( #15533, #4443, #1557, #9354, #10486, #13035, #15442, #12658, #1658, #6562, #276, #11903, #13619, #3795, #4661, #13095 ) ) ;
#12036=CARTESIAN_POINT ( 'NONE',  ( 35.00000000000000000, 50.00000000000000000, 0.000000000000000000 ) ) ;
#12069=DIRECTION ( 'NONE',  ( -0.000000000000000000, 1.000000000000000000, -0.000000000000000000 ) ) ;
#12122=EDGE_LOOP ( 'NONE', ( #8826, #5235, #13372, #14859 ) ) ;
#12134=( NAMED_UNIT ( * ) SI_UNIT ( $, .STERADIAN. ) SOLID_ANGLE_UNIT ( ) );
#12207=SURFACE_SIDE_STYLE ('',( #8527 ) ) ;
#12208=EDGE_CURVE ( 'NONE', #15584, #6071, #13311, .T. ) ;
#12260=DIRECTION ( 'NONE',  ( -0.000000000000000000, 1.000000000000000000, -0.000000000000000000 ) ) ;
#12275=ORIENTED_EDGE ( 'NONE', *, *, #4930, .T. ) ;
#12345=FACE_OUTER_BOUND ( 'NONE', #12122, .T. ) ;
#12346=EDGE_CURVE ( 'NONE', #7943, #11470, #4041, .T. ) ;
#12352=FACE_BOUND ( 'NONE', #8153, .T. ) ;
#12373=ORIENTED_EDGE ( 'NONE', *, *, #13714, .F. ) ;
#12385=UNCERTAINTY_MEASURE_WITH_UNIT (LENGTH_MEASURE( 1.000000000000000082E-05 ), #2512, 'distance_accuracy_value', 'NONE');
#12386=DIRECTION ( 'NONE',  ( 0.000000000000000000, 0.000000000000000000, 1.000000000000000000 ) ) ;
#12394=CARTESIAN_POINT ( 'NONE',  ( -35.00000000000000000, 50.00000000000000000, -2.649999999999985700 ) ) ;
#12441=EDGE_LOOP ( 'NONE', ( #5442, #330, #14186, #1025 ) ) ;
#12519=CIRCLE ( 'NONE', #11750, 2.649999999999985700 ) ;
#12559=ORIENTED_EDGE ( 'NONE', *, *, #186, .T. ) ;
#12612=FACE_OUTER_BOUND ( 'NONE', #6687, .T. ) ;
#12658=ADVANCED_FACE ( 'NONE', ( #6407 ), #10288, .T. ) ;
#12671=DIRECTION ( 'NONE',  ( -0.000000000000000000, 1.000000000000000000, -0.000000000000000000 ) ) ;
#12678=VERTEX_POINT ( 'NONE', #514 ) ;
#12700=LINE ( 'NONE', #9094, #4569 ) ;
#12717=CARTESIAN_POINT ( 'NONE',  ( 67.49999999999931788, 50.00000000000000000, 2.081668171172168513E-14 ) ) ;
#12736=EDGE_LOOP ( 'NONE', ( #15350, #8552 ) ) ;
#12787=DIRECTION ( 'NONE',  ( 0.000000000000000000, 1.000000000000000000, 0.000000000000000000 ) ) ;
#12794=CYLINDRICAL_SURFACE ( 'NONE', #13069, 2.649999999999992806 ) ;
#12801=CARTESIAN_POINT ( 'NONE',  ( -35.00000000000000000, 50.00000000000000000, 2.649999999999992806 ) ) ;
#12818=CYLINDRICAL_SURFACE ( 'NONE', #8950, 2.649999999999985700 ) ;
#12851=PRODUCT_CONTEXT ( 'NONE', #2873, 'mechanical' ) ;
#12899=ORIENTED_EDGE ( 'NONE', *, *, #5413, .F. ) ;
#12935=ORIENTED_EDGE ( 'NONE', *, *, #5062, .F. ) ;
#12972=CARTESIAN_POINT ( 'NONE',  ( -67.50000000000000000, 40.00000000000000000, -7.070249711157346244E-13 ) ) ;
#13035=ADVANCED_FACE ( 'NONE', ( #12345 ), #9607, .F. ) ;
#13038=EDGE_CURVE ( 'NONE', #9472, #4440, #4763, .T. ) ;
#13041=CIRCLE ( 'NONE', #3253, 2.649999999999992806 ) ;
#13042=FACE_OUTER_BOUND ( 'NONE', #6398, .T. ) ;
#13069=AXIS2_PLACEMENT_3D ( 'NONE', #12717, #14018, #13937 ) ;
#13074=ORIENTED_EDGE ( 'NONE', *, *, #934, .F. ) ;
#13095=ADVANCED_FACE ( 'NONE', ( #14625 ), #13546, .F. ) ;
#13110=EDGE_CURVE ( 'NONE', #14412, #2071, #12519, .T. ) ;
#13129=DIRECTION ( 'NONE',  ( 0.000000000000000000, 0.000000000000000000, 1.000000000000000000 ) ) ;
#13137=EDGE_LOOP ( 'NONE', ( #288, #11554 ) ) ;
#13187=ORIENTED_EDGE ( 'NONE', *, *, #15548, .F. ) ;
#13243=CARTESIAN_POINT ( 'NONE',  ( -6.762176242291807225E-13, 50.00000000000000000, 64.84999999999932641 ) ) ;
#13261=VERTEX_POINT ( 'NONE', #9523 ) ;
#13280=EDGE_CURVE ( 'NONE', #4993, #6462, #13041, .T. ) ;
#13287=CARTESIAN_POINT ( 'NONE',  ( 0.000000000000000000, 40.00000000000000000, 0.000000000000000000 ) ) ;
#13308=AXIS2_PLACEMENT_3D ( 'NONE', #5766, #15640, #11821 ) ;
#13311=CIRCLE ( 'NONE', #14885, 2.649999999999985700 ) ;
#13314=DIRECTION ( 'NONE',  ( 0.000000000000000000, 1.000000000000000000, 0.000000000000000000 ) ) ;
#13372=ORIENTED_EDGE ( 'NONE', *, *, #12346, .T. ) ;
#13379=FACE_OUTER_BOUND ( 'NONE', #8845, .T. ) ;
#13406=CARTESIAN_POINT ( 'NONE',  ( 2.143131898507869826E-15, 40.00000000000000000, -67.50000000000000000 ) ) ;
#13414=EDGE_CURVE ( 'NONE', #1037, #10616, #3472, .T. ) ;
#13437=CARTESIAN_POINT ( 'NONE',  ( -6.762176242291807225E-13, 50.00000000000000000, 64.84999999999932641 ) ) ;
#13504=CARTESIAN_POINT ( 'NONE',  ( -35.00000000000000000, 40.00000000000000000, 0.000000000000000000 ) ) ;
#13523=CARTESIAN_POINT ( 'NONE',  ( 2.467663300281918521E-15, 40.00000000000000000, -70.14999999999999147 ) ) ;
#13546=CYLINDRICAL_SURFACE ( 'NONE', #12003, 2.649999999999992806 ) ;
#13582=PRESENTATION_STYLE_ASSIGNMENT (( #14569 ) ) ;
#13602=ORIENTED_EDGE ( 'NONE', *, *, #2102, .F. ) ;
#13607=DIRECTION ( 'NONE',  ( -0.000000000000000000, 1.000000000000000000, -0.000000000000000000 ) ) ;
#13613=CARTESIAN_POINT ( 'NONE',  ( -35.00000000000000000, 50.00000000000000000, 0.000000000000000000 ) ) ;
#13619=ADVANCED_FACE ( 'NONE', ( #9997 ), #14933, .F. ) ;
#13632=ORIENTED_EDGE ( 'NONE', *, *, #1343, .F. ) ;
#13636=CARTESIAN_POINT ( 'NONE',  ( -6.765421556309547668E-13, 40.00000000000000000, 67.49999999999930367 ) ) ;
#13646=CARTESIAN_POINT ( 'NONE',  ( -6.765421556309547668E-13, 40.00000000000000000, 70.14999999999929514 ) ) ;
#13651=EDGE_LOOP ( 'NONE', ( #2534, #5768 ) ) ;
#13668=FILL_AREA_STYLE ('',( #3821 ) ) ;
#13678=LINE ( 'NONE', #3981, #3021 ) ;
#13697=CARTESIAN_POINT ( 'NONE',  ( -67.50000000000000000, 50.00000000000000000, -7.070249711157346244E-13 ) ) ;
#13714=EDGE_CURVE ( 'NONE', #10675, #15345, #5796, .T. ) ;
#13722=CARTESIAN_POINT ( 'NONE',  ( -67.50000000000000000, 50.00000000000000000, -2.650000000000699352 ) ) ;
#13757=DIRECTION ( 'NONE',  ( -0.000000000000000000, 1.000000000000000000, -0.000000000000000000 ) ) ;
#13813=VECTOR ( 'NONE', #12671, 1000.000000000000000 ) ;
#13850=AXIS2_PLACEMENT_3D ( 'NONE', #15256, #5704, #4247 ) ;
#13900=ORIENTED_EDGE ( 'NONE', *, *, #14393, .T. ) ;
#13915=VERTEX_POINT ( 'NONE', #15880 ) ;
#13937=DIRECTION ( 'NONE',  ( 0.000000000000000000, 0.000000000000000000, 1.000000000000000000 ) ) ;
#14018=DIRECTION ( 'NONE',  ( -0.000000000000000000, 1.000000000000000000, -0.000000000000000000 ) ) ;
#14034=UNCERTAINTY_MEASURE_WITH_UNIT (LENGTH_MEASURE( 1.000000000000000082E-05 ), #2199, 'distance_accuracy_value', 'NONE');
#14035=FACE_OUTER_BOUND ( 'NONE', #12441, .T. ) ;
#14094=AXIS2_PLACEMENT_3D ( 'NONE', #13636, #2726, #11217 ) ;
#14111=DIRECTION ( 'NONE',  ( 0.000000000000000000, 1.000000000000000000, 0.000000000000000000 ) ) ;
#14159=AXIS2_PLACEMENT_3D ( 'NONE', #5454, #613, #1806 ) ;
#14181=DIRECTION ( 'NONE',  ( -0.000000000000000000, -1.000000000000000000, -0.000000000000000000 ) ) ;
#14186=ORIENTED_EDGE ( 'NONE', *, *, #11988, .T. ) ;
#14263=ORIENTED_EDGE ( 'NONE', *, *, #13414, .T. ) ;
#14308=ORIENTED_EDGE ( 'NONE', *, *, #13414, .F. ) ;
#14323=STYLED_ITEM ( 'NONE', ( #13582 ), #6582 ) ;
#14324=AXIS2_PLACEMENT_3D ( 'NONE', #12036, #2181, #4772 ) ;
#14384=CARTESIAN_POINT ( 'NONE',  ( 9.184850993605153466E-15, 50.00000000000000000, 75.00000000000004263 ) ) ;
#14393=EDGE_CURVE ( 'NONE', #3118, #15938, #8924, .T. ) ;
#14411=EDGE_CURVE ( 'NONE', #11470, #7943, #14845, .T. ) ;
#14412=VERTEX_POINT ( 'NONE', #13243 ) ;
#14453=DIRECTION ( 'NONE',  ( 0.000000000000000000, 0.000000000000000000, 1.000000000000000000 ) ) ;
#14492=PRESENTATION_STYLE_ASSIGNMENT (( #7233 ) ) ;
#14543=CARTESIAN_POINT ( 'NONE',  ( 67.49999999999931788, 50.00000000000000000, 2.081668171172168513E-14 ) ) ;
#14569=SURFACE_STYLE_USAGE ( .BOTH. , #3732 ) ;
#14579=CIRCLE ( 'NONE', #8143, 2.649999999999985700 ) ;
#14592=VERTEX_POINT ( 'NONE', #3641 ) ;
#14603=CARTESIAN_POINT ( 'NONE',  ( 0.000000000000000000, 50.00000000000000000, 0.000000000000000000 ) ) ;
#14620=EDGE_CURVE ( 'NONE', #13915, #4440, #14579, .T. ) ;
#14625=FACE_OUTER_BOUND ( 'NONE', #15142, .T. ) ;
#14635=CARTESIAN_POINT ( 'NONE',  ( 67.49999999999931788, 50.00000000000000000, 2.081668171172168513E-14 ) ) ;
#14639=ORIENTED_EDGE ( 'NONE', *, *, #14411, .T. ) ;
#14653=CIRCLE ( 'NONE', #7707, 2.649999999999985700 ) ;
#14672=EDGE_CURVE ( 'NONE', #12016, #12678, #1147, .T. ) ;
#14744=DIRECTION ( 'NONE',  ( 0.000000000000000000, 1.000000000000000000, 0.000000000000000000 ) ) ;
#14755=CIRCLE ( 'NONE', #3651, 2.649999999999992806 ) ;
#14818=EDGE_CURVE ( 'NONE', #4993, #7943, #1369, .T. ) ;
#14823=CARTESIAN_POINT ( 'NONE',  ( 67.49999999999931788, 40.00000000000000000, -2.649999999999971934 ) ) ;
#14833=AXIS2_PLACEMENT_3D ( 'NONE', #1896, #14111, #15411 ) ;
#14845=CIRCLE ( 'NONE', #1417, 2.649999999999985700 ) ;
#14859=ORIENTED_EDGE ( 'NONE', *, *, #5097, .F. ) ;
#14861=CARTESIAN_POINT ( 'NONE',  ( -67.50000000000000000, 40.00000000000000000, -2.650000000000699352 ) ) ;
#14870=AXIS2_PLACEMENT_3D ( 'NONE', #13287, #10958, #9589 ) ;
#14885=AXIS2_PLACEMENT_3D ( 'NONE', #13613, #11122, #3923 ) ;
#14933=CYLINDRICAL_SURFACE ( 'NONE', #10708, 2.649999999999992806 ) ;
#14990=EDGE_CURVE ( 'NONE', #14592, #9703, #9188, .T. ) ;
#15043=ORIENTED_EDGE ( 'NONE', *, *, #8630, .T. ) ;
#15095=ORIENTED_EDGE ( 'NONE', *, *, #13110, .F. ) ;
#15142=EDGE_LOOP ( 'NONE', ( #12899, #12373, #7859, #15043 ) ) ;
#15219=DIRECTION ( 'NONE',  ( 0.000000000000000000, 0.000000000000000000, 1.000000000000000000 ) ) ;
#15256=CARTESIAN_POINT ( 'NONE',  ( -35.00000000000000000, 50.00000000000000000, 0.000000000000000000 ) ) ;
#15268=EDGE_LOOP ( 'NONE', ( #15724, #8195, #2835, #14263 ) ) ;
#15289=EDGE_CURVE ( 'NONE', #9472, #10300, #4023, .T. ) ;
#15334=DIRECTION ( 'NONE',  ( -0.000000000000000000, 1.000000000000000000, -0.000000000000000000 ) ) ;
#15345=VERTEX_POINT ( 'NONE', #15427 ) ;
#15350=ORIENTED_EDGE ( 'NONE', *, *, #13714, .T. ) ;
#15359=DIRECTION ( 'NONE',  ( -0.000000000000000000, 1.000000000000000000, -0.000000000000000000 ) ) ;
#15365=ORIENTED_EDGE ( 'NONE', *, *, #12346, .F. ) ;
#15373=( GEOMETRIC_REPRESENTATION_CONTEXT ( 3 ) GLOBAL_UNCERTAINTY_ASSIGNED_CONTEXT ( ( #11265 ) ) GLOBAL_UNIT_ASSIGNED_CONTEXT ( ( #1071, #37, #12134 ) ) REPRESENTATION_CONTEXT ( 'NONE', 'WORKASPACE' ) );
#15411=DIRECTION ( 'NONE',  ( 0.000000000000000000, 0.000000000000000000, 1.000000000000000000 ) ) ;
#15427=CARTESIAN_POINT ( 'NONE',  ( 35.00000000000000000, 40.00000000000000000, -2.649999999999992806 ) ) ;
#15433=DIRECTION ( 'NONE',  ( -0.000000000000000000, 1.000000000000000000, -0.000000000000000000 ) ) ;
#15442=ADVANCED_FACE ( 'NONE', ( #14035 ), #2960, .T. ) ;
#15447=CARTESIAN_POINT ( 'NONE',  ( 35.00000000000000000, 50.00000000000000000, 0.000000000000000000 ) ) ;
#15489=CARTESIAN_POINT ( 'NONE',  ( -6.765421556309547668E-13, 50.00000000000000000, 67.49999999999930367 ) ) ;
#15533=ADVANCED_FACE ( 'NONE', ( #8154 ), #11845, .F. ) ;
#15541=DIRECTION ( 'NONE',  ( 0.000000000000000000, 0.000000000000000000, 1.000000000000000000 ) ) ;
#15548=EDGE_CURVE ( 'NONE', #3191, #15584, #6355, .T. ) ;
#15584=VERTEX_POINT ( 'NONE', #12394 ) ;
#15591=CARTESIAN_POINT ( 'NONE',  ( 2.143131898507869826E-15, 50.00000000000000000, -67.50000000000000000 ) ) ;
#15640=DIRECTION ( 'NONE',  ( -0.000000000000000000, 1.000000000000000000, -0.000000000000000000 ) ) ;
#15678=DIRECTION ( 'NONE',  ( 0.000000000000000000, 0.000000000000000000, 1.000000000000000000 ) ) ;
#15682=DIRECTION ( 'NONE',  ( 0.000000000000000000, 1.000000000000000000, 0.000000000000000000 ) ) ;
#15691=EDGE_CURVE ( 'NONE', #13261, #14412, #54, .T. ) ;
#15724=ORIENTED_EDGE ( 'NONE', *, *, #5825, .F. ) ;
#15746=DIRECTION ( 'NONE',  ( 0.000000000000000000, 0.000000000000000000, -1.000000000000000000 ) ) ;
#15756=PLANE ( 'NONE',  #1866 ) ;
#15782=ORIENTED_EDGE ( 'NONE', *, *, #11650, .F. ) ;
#15793=( NAMED_UNIT ( * ) PLANE_ANGLE_UNIT ( ) SI_UNIT ( $, .RADIAN. ) );
#15807=DIRECTION ( 'NONE',  ( 0.000000000000000000, 1.000000000000000000, 0.000000000000000000 ) ) ;
#15814=EDGE_CURVE ( 'NONE', #9703, #14592, #8406, .T. ) ;
#15818=CARTESIAN_POINT ( 'NONE',  ( 35.00000000000000000, 50.00000000000000000, 0.000000000000000000 ) ) ;
#15839=EDGE_LOOP ( 'NONE', ( #3703, #10846, #323, #12935 ) ) ;
#15880=CARTESIAN_POINT ( 'NONE',  ( -67.50000000000000000, 50.00000000000000000, -2.650000000000692690 ) ) ;
#15909=VECTOR ( 'NONE', #13607, 1000.000000000000000 ) ;
#15933=AXIS2_PLACEMENT_3D ( 'NONE', #9998, #1338, #8954 ) ;
#15938=VERTEX_POINT ( 'NONE', #1003 ) ;
#15960=CIRCLE ( 'NONE', #5895, 2.649999999999992806 ) ;
#15961=AXIS2_PLACEMENT_3D ( 'NONE', #11143, #13314, #1121 ) ;
ENDSEC;
END-ISO-10303-21;
